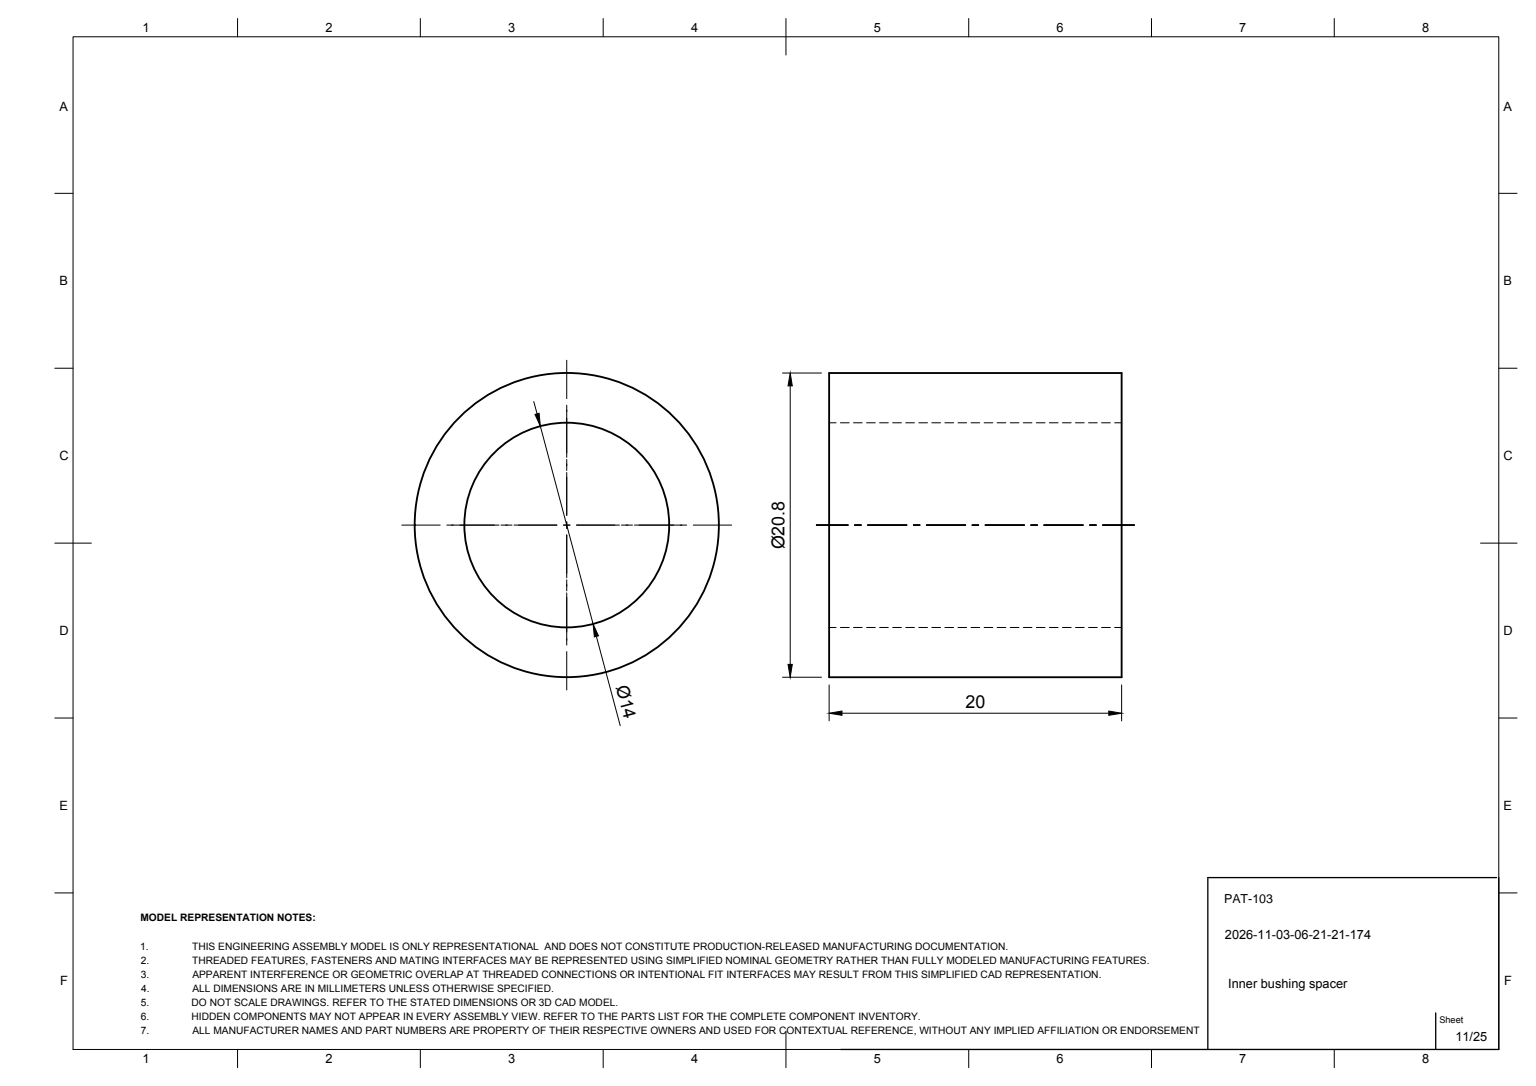
ISO-10303-21;
HEADER;
/* Generated by software containing ST-Developer
 * from STEP Tools, Inc. (www.steptools.com) 
 */

FILE_DESCRIPTION(
/* description */ ('Telescoping shaft support with lock collar'),
/* implementation_level */ '2;1');

FILE_NAME(
/* name */ 'Inner bushing spacer.step',
/* time_stamp */ '2026-10-27T10:48:51-07:00',
/* author */ (''),
/* organization */ (''),
/* preprocessor_version */ 'ST-DEVELOPER v20.2',
/* originating_system */ 'Autodesk Translation Framework v15.17.0.0',
/* authorisation */ '');

FILE_SCHEMA (('AUTOMOTIVE_DESIGN { 1 0 10303 214 3 1 1 }'));
ENDSEC;

DATA;
#10=MECHANICAL_DESIGN_GEOMETRIC_PRESENTATION_REPRESENTATION('',(#247),#7349);
#207=SHAPE_REPRESENTATION_RELATIONSHIP('SRR','None',#7449,#227);
#227=ADVANCED_BREP_SHAPE_REPRESENTATION('',(#267),#7333);
#247=STYLED_ITEM('',(#7620),#267);
#267=MANIFOLD_SOLID_BREP('Body1',#3970);
#313=FACE_BOUND('',#848,.T.);
#314=FACE_BOUND('',#850,.T.);
#415=PLANE('',#4404);
#416=PLANE('',#4405);
#585=FACE_OUTER_BOUND('',#845,.T.);
#586=FACE_OUTER_BOUND('',#846,.T.);
#587=FACE_OUTER_BOUND('',#847,.T.);
#588=FACE_OUTER_BOUND('',#849,.T.);
#845=EDGE_LOOP('',(#3086,#3087,#3088,#3089));
#846=EDGE_LOOP('',(#3090,#3091,#3092,#3093));
#847=EDGE_LOOP('',(#3094));
#848=EDGE_LOOP('',(#3095));
#849=EDGE_LOOP('',(#3096));
#850=EDGE_LOOP('',(#3097));
#1157=LINE('',#6460,#1437);
#1158=LINE('',#6466,#1438);
#1437=VECTOR('',#5223,0.7);
#1438=VECTOR('',#5230,1.04);
#1679=CIRCLE('',#4399,0.7);
#1680=CIRCLE('',#4400,0.7);
#1681=CIRCLE('',#4402,1.04);
#1682=CIRCLE('',#4403,1.04);
#1946=VERTEX_POINT('',#6457);
#1947=VERTEX_POINT('',#6459);
#1948=VERTEX_POINT('',#6463);
#1949=VERTEX_POINT('',#6465);
#2355=EDGE_CURVE('',#1946,#1946,#1679,.T.);
#2356=EDGE_CURVE('',#1946,#1947,#1157,.T.);
#2357=EDGE_CURVE('',#1947,#1947,#1680,.T.);
#2358=EDGE_CURVE('',#1948,#1948,#1681,.T.);
#2359=EDGE_CURVE('',#1948,#1949,#1158,.T.);
#2360=EDGE_CURVE('',#1949,#1949,#1682,.T.);
#3086=ORIENTED_EDGE('',*,*,#2355,.F.);
#3087=ORIENTED_EDGE('',*,*,#2356,.T.);
#3088=ORIENTED_EDGE('',*,*,#2357,.T.);
#3089=ORIENTED_EDGE('',*,*,#2356,.F.);
#3090=ORIENTED_EDGE('',*,*,#2358,.F.);
#3091=ORIENTED_EDGE('',*,*,#2359,.T.);
#3092=ORIENTED_EDGE('',*,*,#2360,.T.);
#3093=ORIENTED_EDGE('',*,*,#2359,.F.);
#3094=ORIENTED_EDGE('',*,*,#2358,.T.);
#3095=ORIENTED_EDGE('',*,*,#2355,.T.);
#3096=ORIENTED_EDGE('',*,*,#2360,.F.);
#3097=ORIENTED_EDGE('',*,*,#2357,.F.);
#3694=CYLINDRICAL_SURFACE('',#4398,0.7);
#3695=CYLINDRICAL_SURFACE('',#4401,1.04);
#3828=ADVANCED_FACE('',(#585),#3694,.F.);
#3829=ADVANCED_FACE('',(#586),#3695,.T.);
#3830=ADVANCED_FACE('',(#587,#313),#415,.T.);
#3831=ADVANCED_FACE('',(#588,#314),#416,.F.);
#3970=CLOSED_SHELL('',(#3828,#3829,#3830,#3831));
#4397=AXIS2_PLACEMENT_3D('',#6455,#5217,#5218);
#4398=AXIS2_PLACEMENT_3D('',#6456,#5219,#5220);
#4399=AXIS2_PLACEMENT_3D('',#6458,#5221,#5222);
#4400=AXIS2_PLACEMENT_3D('',#6461,#5224,#5225);
#4401=AXIS2_PLACEMENT_3D('',#6462,#5226,#5227);
#4402=AXIS2_PLACEMENT_3D('',#6464,#5228,#5229);
#4403=AXIS2_PLACEMENT_3D('',#6467,#5231,#5232);
#4404=AXIS2_PLACEMENT_3D('',#6468,#5233,#5234);
#4405=AXIS2_PLACEMENT_3D('',#6469,#5235,#5236);
#5217=DIRECTION('axis',(0.,0.,1.));
#5218=DIRECTION('refdir',(1.,0.,0.));
#5219=DIRECTION('center_axis',(1.,0.,0.));
#5220=DIRECTION('ref_axis',(0.,0.,-1.));
#5221=DIRECTION('center_axis',(-1.,0.,0.));
#5222=DIRECTION('ref_axis',(0.,0.,-1.));
#5223=DIRECTION('',(-1.,0.,0.));
#5224=DIRECTION('center_axis',(-1.,0.,0.));
#5225=DIRECTION('ref_axis',(0.,0.,-1.));
#5226=DIRECTION('center_axis',(1.,0.,0.));
#5227=DIRECTION('ref_axis',(0.,0.,-1.));
#5228=DIRECTION('center_axis',(1.,0.,0.));
#5229=DIRECTION('ref_axis',(0.,0.,-1.));
#5230=DIRECTION('',(-1.,0.,0.));
#5231=DIRECTION('center_axis',(1.,0.,0.));
#5232=DIRECTION('ref_axis',(0.,0.,-1.));
#5233=DIRECTION('center_axis',(1.,0.,0.));
#5234=DIRECTION('ref_axis',(0.,0.,-1.));
#5235=DIRECTION('center_axis',(1.,0.,0.));
#5236=DIRECTION('ref_axis',(0.,0.,-1.));
#6455=CARTESIAN_POINT('',(0.,0.,0.));
#6456=CARTESIAN_POINT('Origin',(4.,0.,3.5));
#6457=CARTESIAN_POINT('',(6.,-8.57252759403147E-17,4.2));
#6458=CARTESIAN_POINT('Origin',(6.,0.,3.5));
#6459=CARTESIAN_POINT('',(4.,-8.57252759403147E-17,4.2));
#6460=CARTESIAN_POINT('',(4.,-8.57252759403147E-17,4.2));
#6461=CARTESIAN_POINT('Origin',(4.,0.,3.5));
#6462=CARTESIAN_POINT('Origin',(4.,0.,3.5));
#6463=CARTESIAN_POINT('',(6.,-1.27363267111325E-16,4.54));
#6464=CARTESIAN_POINT('Origin',(6.,0.,3.5));
#6465=CARTESIAN_POINT('',(4.,-1.27363267111325E-16,4.54));
#6466=CARTESIAN_POINT('',(4.,-1.27363267111325E-16,4.54));
#6467=CARTESIAN_POINT('Origin',(4.,0.,3.5));
#6468=CARTESIAN_POINT('Origin',(6.,0.,3.5));
#6469=CARTESIAN_POINT('Origin',(4.,0.,3.5));
#7308=UNCERTAINTY_MEASURE_WITH_UNIT(LENGTH_MEASURE(0.001),#7350,
'DISTANCE_ACCURACY_VALUE',
'Maximum model space distance between geometric entities at asserted c
onnectivities');
#7324=UNCERTAINTY_MEASURE_WITH_UNIT(LENGTH_MEASURE(0.001),#7350,
'DISTANCE_ACCURACY_VALUE',
'Maximum model space distance between geometric entities at asserted c
onnectivities');
#7333=(
GEOMETRIC_REPRESENTATION_CONTEXT(3)
GLOBAL_UNCERTAINTY_ASSIGNED_CONTEXT((#7308))
GLOBAL_UNIT_ASSIGNED_CONTEXT((#7350,#7352,#7353))
REPRESENTATION_CONTEXT('','3D')
);
#7349=(
GEOMETRIC_REPRESENTATION_CONTEXT(3)
GLOBAL_UNCERTAINTY_ASSIGNED_CONTEXT((#7324))
GLOBAL_UNIT_ASSIGNED_CONTEXT((#7350,#7352,#7353))
REPRESENTATION_CONTEXT('','3D')
);
#7350=(
LENGTH_UNIT()
NAMED_UNIT(*)
SI_UNIT(.CENTI.,.METRE.)
);
#7352=(
NAMED_UNIT(*)
PLANE_ANGLE_UNIT()
SI_UNIT($,.RADIAN.)
);
#7353=(
NAMED_UNIT(*)
SI_UNIT($,.STERADIAN.)
SOLID_ANGLE_UNIT()
);
#7362=SHAPE_DEFINITION_REPRESENTATION(#7386,#7449);
#7386=PRODUCT_DEFINITION_SHAPE('',$,#7474);
#7449=SHAPE_REPRESENTATION('',(#4397),#7333);
#7465=PRODUCT_DEFINITION_CONTEXT('part definition',#7539,'design');
#7474=PRODUCT_DEFINITION('Inner bushing spacer','Inner bushing spacer',
#7498,#7465);
#7498=PRODUCT_DEFINITION_FORMATION('',$,#7549);
#7539=APPLICATION_CONTEXT(
'Core Data for Automotive Mechanical Design Process');
#7540=PRODUCT_CONTEXT('part definition',#7539,'mechanical');
#7549=PRODUCT('Inner bushing spacer','Inner bushing spacer',
'Inner bushing spacer',(#7540));
#7614=COLOUR_RGB('Sky Blue',0.24,0.69,0.87);
#7615=FILL_AREA_STYLE_COLOUR('',#7614);
#7616=FILL_AREA_STYLE('',(#7615));
#7617=SURFACE_STYLE_FILL_AREA(#7616);
#7618=SURFACE_SIDE_STYLE('',(#7617));
#7619=SURFACE_STYLE_USAGE(.BOTH.,#7618);
#7620=PRESENTATION_STYLE_ASSIGNMENT((#7619));
ENDSEC;
END-ISO-10303-21;
